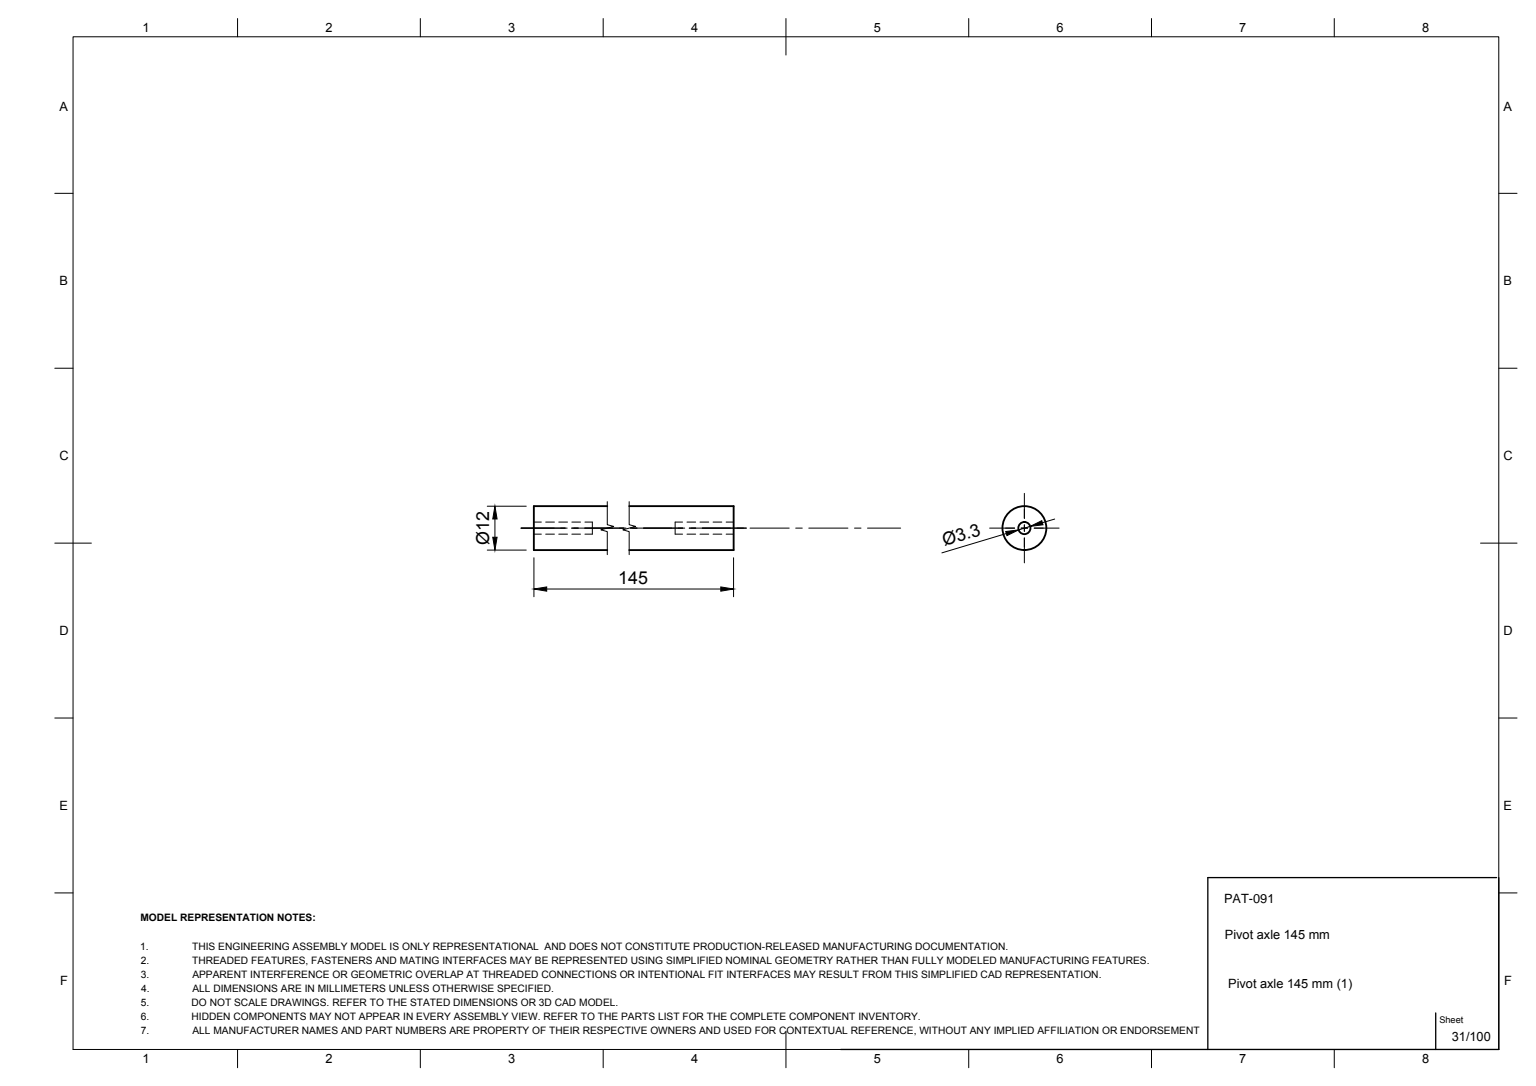
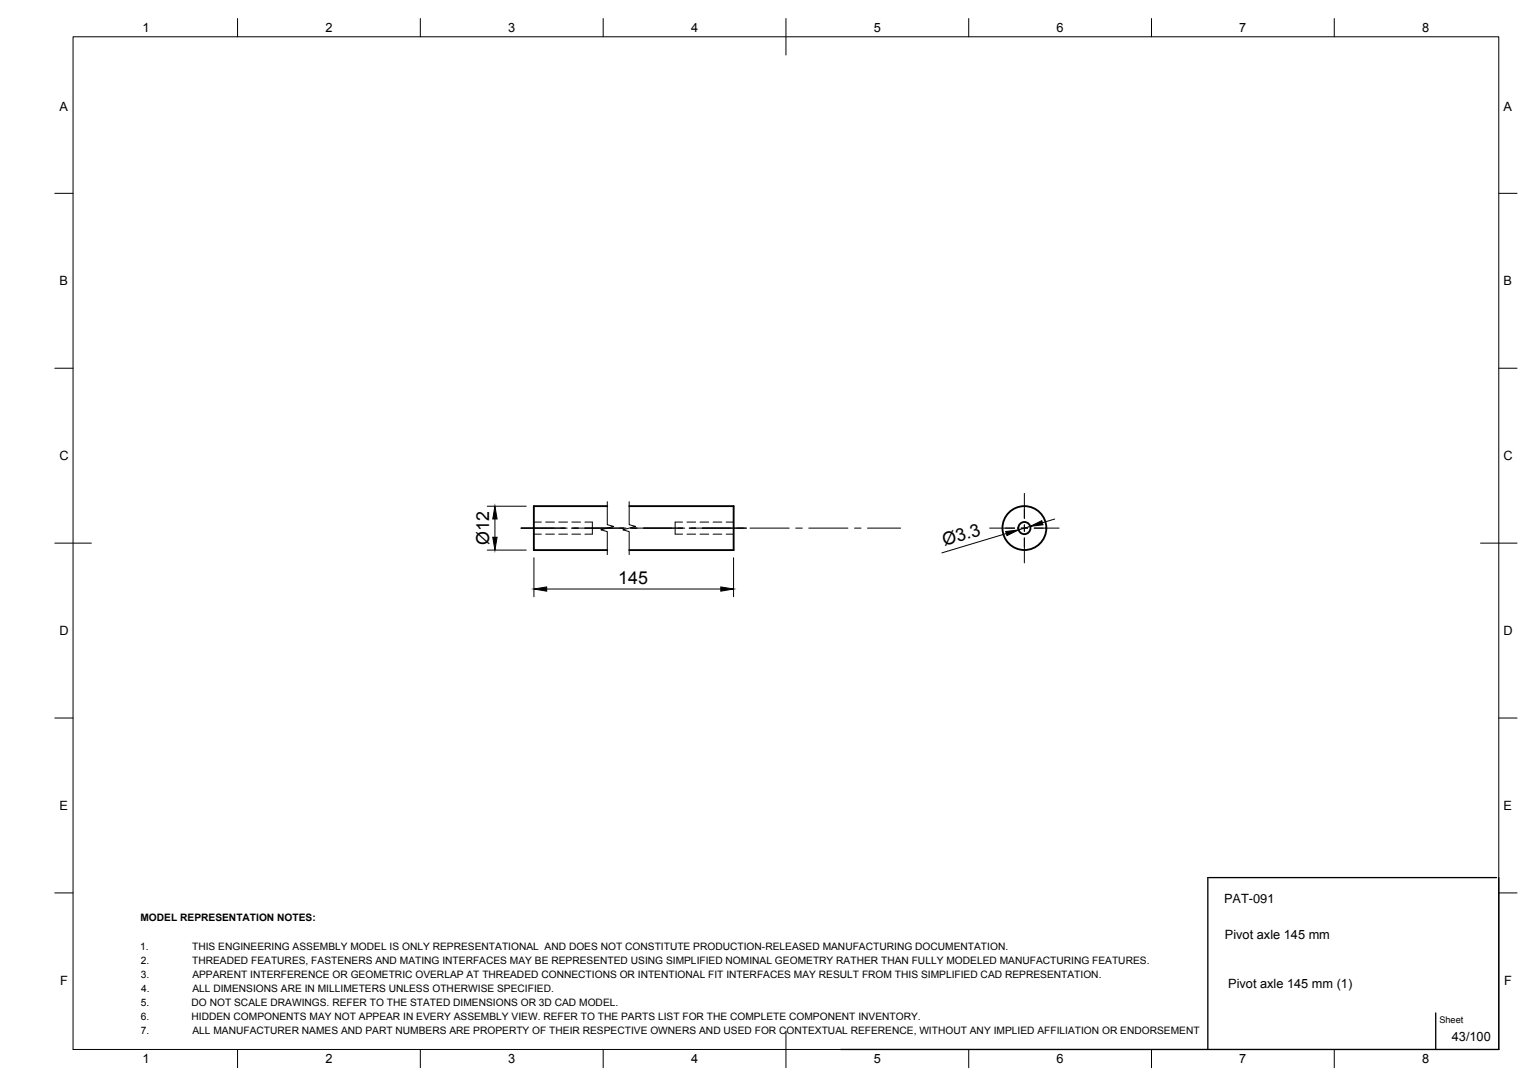
ISO-10303-21;
HEADER;
/* Generated by software containing ST-Developer
 * from STEP Tools, Inc. (www.steptools.com) 
 */

FILE_DESCRIPTION(
/* description */ ('PAT-091'),
/* implementation_level */ '2;1');

FILE_NAME(
/* name */ 'Pivot axle 145 mm.step',
/* time_stamp */ '2026-10-27T15:34:44-07:00',
/* author */ (''),
/* organization */ (''),
/* preprocessor_version */ 'ST-DEVELOPER v20.2',
/* originating_system */ 'Autodesk Translation Framework v15.17.0.0',
/* authorisation */ '');

FILE_SCHEMA (('AUTOMOTIVE_DESIGN { 1 0 10303 214 3 1 1 }'));
ENDSEC;

DATA;
#10=MECHANICAL_DESIGN_GEOMETRIC_PRESENTATION_REPRESENTATION('',(#994),#25100);
#774=SHAPE_REPRESENTATION_RELATIONSHIP('SRR','None',#25536,#884);
#884=ADVANCED_BREP_SHAPE_REPRESENTATION('',(#1117),#25006);
#994=STYLED_ITEM('',(#26191),#1117);
#1117=MANIFOLD_SOLID_BREP('Body1',#13272);
#1377=FACE_BOUND('',#3261,.T.);
#1378=FACE_BOUND('',#3263,.T.);
#1750=PLANE('',#15028);
#1751=PLANE('',#15032);
#1752=PLANE('',#15036);
#1753=PLANE('',#15037);
#2275=FACE_OUTER_BOUND('',#3255,.T.);
#2276=FACE_OUTER_BOUND('',#3256,.T.);
#2277=FACE_OUTER_BOUND('',#3257,.T.);
#2278=FACE_OUTER_BOUND('',#3258,.T.);
#2279=FACE_OUTER_BOUND('',#3259,.T.);
#2280=FACE_OUTER_BOUND('',#3260,.T.);
#2281=FACE_OUTER_BOUND('',#3262,.T.);
#3255=EDGE_LOOP('',(#9902,#9903,#9904,#9905));
#3256=EDGE_LOOP('',(#9906));
#3257=EDGE_LOOP('',(#9907,#9908,#9909,#9910));
#3258=EDGE_LOOP('',(#9911));
#3259=EDGE_LOOP('',(#9912,#9913,#9914,#9915));
#3260=EDGE_LOOP('',(#9916));
#3261=EDGE_LOOP('',(#9917));
#3262=EDGE_LOOP('',(#9918));
#3263=EDGE_LOOP('',(#9919));
#4388=LINE('',#21991,#5128);
#4389=LINE('',#21998,#5129);
#4390=LINE('',#22005,#5130);
#5128=VECTOR('',#17616,0.165);
#5129=VECTOR('',#17625,0.165);
#5130=VECTOR('',#17634,0.6);
#5805=CIRCLE('',#15026,0.165);
#5806=CIRCLE('',#15027,0.165);
#5807=CIRCLE('',#15030,0.165);
#5808=CIRCLE('',#15031,0.165);
#5809=CIRCLE('',#15034,0.6);
#5810=CIRCLE('',#15035,0.6);
#6692=VERTEX_POINT('',#21988);
#6693=VERTEX_POINT('',#21990);
#6694=VERTEX_POINT('',#21995);
#6695=VERTEX_POINT('',#21997);
#6696=VERTEX_POINT('',#22002);
#6697=VERTEX_POINT('',#22004);
#7886=EDGE_CURVE('',#6692,#6692,#5805,.T.);
#7887=EDGE_CURVE('',#6692,#6693,#4388,.T.);
#7888=EDGE_CURVE('',#6693,#6693,#5806,.T.);
#7889=EDGE_CURVE('',#6694,#6694,#5807,.T.);
#7890=EDGE_CURVE('',#6694,#6695,#4389,.T.);
#7891=EDGE_CURVE('',#6695,#6695,#5808,.T.);
#7892=EDGE_CURVE('',#6696,#6696,#5809,.T.);
#7893=EDGE_CURVE('',#6696,#6697,#4390,.T.);
#7894=EDGE_CURVE('',#6697,#6697,#5810,.T.);
#9902=ORIENTED_EDGE('',*,*,#7886,.F.);
#9903=ORIENTED_EDGE('',*,*,#7887,.T.);
#9904=ORIENTED_EDGE('',*,*,#7888,.F.);
#9905=ORIENTED_EDGE('',*,*,#7887,.F.);
#9906=ORIENTED_EDGE('',*,*,#7886,.T.);
#9907=ORIENTED_EDGE('',*,*,#7889,.F.);
#9908=ORIENTED_EDGE('',*,*,#7890,.T.);
#9909=ORIENTED_EDGE('',*,*,#7891,.T.);
#9910=ORIENTED_EDGE('',*,*,#7890,.F.);
#9911=ORIENTED_EDGE('',*,*,#7891,.F.);
#9912=ORIENTED_EDGE('',*,*,#7892,.F.);
#9913=ORIENTED_EDGE('',*,*,#7893,.T.);
#9914=ORIENTED_EDGE('',*,*,#7894,.T.);
#9915=ORIENTED_EDGE('',*,*,#7893,.F.);
#9916=ORIENTED_EDGE('',*,*,#7892,.T.);
#9917=ORIENTED_EDGE('',*,*,#7888,.T.);
#9918=ORIENTED_EDGE('',*,*,#7894,.F.);
#9919=ORIENTED_EDGE('',*,*,#7889,.T.);
#12173=CYLINDRICAL_SURFACE('',#15025,0.165);
#12174=CYLINDRICAL_SURFACE('',#15029,0.165);
#12175=CYLINDRICAL_SURFACE('',#15033,0.6);
#12642=ADVANCED_FACE('',(#2275),#12173,.F.);
#12643=ADVANCED_FACE('',(#2276),#1750,.T.);
#12644=ADVANCED_FACE('',(#2277),#12174,.F.);
#12645=ADVANCED_FACE('',(#2278),#1751,.F.);
#12646=ADVANCED_FACE('',(#2279),#12175,.T.);
#12647=ADVANCED_FACE('',(#2280,#1377),#1752,.T.);
#12648=ADVANCED_FACE('',(#2281,#1378),#1753,.F.);
#13272=CLOSED_SHELL('',(#12642,#12643,#12644,#12645,#12646,#12647,#12648));
#15024=AXIS2_PLACEMENT_3D('',#21986,#17610,#17611);
#15025=AXIS2_PLACEMENT_3D('',#21987,#17612,#17613);
#15026=AXIS2_PLACEMENT_3D('',#21989,#17614,#17615);
#15027=AXIS2_PLACEMENT_3D('',#21992,#17617,#17618);
#15028=AXIS2_PLACEMENT_3D('',#21993,#17619,#17620);
#15029=AXIS2_PLACEMENT_3D('',#21994,#17621,#17622);
#15030=AXIS2_PLACEMENT_3D('',#21996,#17623,#17624);
#15031=AXIS2_PLACEMENT_3D('',#21999,#17626,#17627);
#15032=AXIS2_PLACEMENT_3D('',#22000,#17628,#17629);
#15033=AXIS2_PLACEMENT_3D('',#22001,#17630,#17631);
#15034=AXIS2_PLACEMENT_3D('',#22003,#17632,#17633);
#15035=AXIS2_PLACEMENT_3D('',#22006,#17635,#17636);
#15036=AXIS2_PLACEMENT_3D('',#22007,#17637,#17638);
#15037=AXIS2_PLACEMENT_3D('',#22008,#17639,#17640);
#17610=DIRECTION('axis',(0.,0.,1.));
#17611=DIRECTION('refdir',(1.,0.,0.));
#17612=DIRECTION('center_axis',(0.,1.,0.));
#17613=DIRECTION('ref_axis',(1.,0.,0.));
#17614=DIRECTION('center_axis',(0.,1.,0.));
#17615=DIRECTION('ref_axis',(1.,0.,0.));
#17616=DIRECTION('',(0.,1.,0.));
#17617=DIRECTION('center_axis',(0.,-1.,0.));
#17618=DIRECTION('ref_axis',(1.,0.,0.));
#17619=DIRECTION('center_axis',(0.,1.,0.));
#17620=DIRECTION('ref_axis',(1.,0.,0.));
#17621=DIRECTION('center_axis',(0.,1.,0.));
#17622=DIRECTION('ref_axis',(1.,0.,0.));
#17623=DIRECTION('center_axis',(0.,1.,0.));
#17624=DIRECTION('ref_axis',(1.,0.,0.));
#17625=DIRECTION('',(0.,1.,0.));
#17626=DIRECTION('center_axis',(0.,1.,0.));
#17627=DIRECTION('ref_axis',(1.,0.,0.));
#17628=DIRECTION('center_axis',(0.,1.,0.));
#17629=DIRECTION('ref_axis',(1.,0.,0.));
#17630=DIRECTION('center_axis',(0.,1.,0.));
#17631=DIRECTION('ref_axis',(1.,0.,0.));
#17632=DIRECTION('center_axis',(0.,1.,0.));
#17633=DIRECTION('ref_axis',(1.,0.,0.));
#17634=DIRECTION('',(0.,-1.,0.));
#17635=DIRECTION('center_axis',(0.,1.,0.));
#17636=DIRECTION('ref_axis',(1.,0.,0.));
#17637=DIRECTION('center_axis',(0.,1.,0.));
#17638=DIRECTION('ref_axis',(1.,0.,0.));
#17639=DIRECTION('center_axis',(0.,1.,0.));
#17640=DIRECTION('ref_axis',(1.,0.,0.));
#21986=CARTESIAN_POINT('',(0.,0.,0.));
#21987=CARTESIAN_POINT('Origin',(0.,6.9,13.));
#21988=CARTESIAN_POINT('',(-0.165,6.9,13.));
#21989=CARTESIAN_POINT('Origin',(0.,6.9,13.));
#21990=CARTESIAN_POINT('',(-0.165,8.5,13.));
#21991=CARTESIAN_POINT('',(-0.165,6.9,13.));
#21992=CARTESIAN_POINT('Origin',(0.,8.5,13.));
#21993=CARTESIAN_POINT('Origin',(0.,6.9,13.));
#21994=CARTESIAN_POINT('Origin',(0.,-6.1,13.));
#21995=CARTESIAN_POINT('',(-0.165,-6.,13.));
#21996=CARTESIAN_POINT('Origin',(0.,-6.,13.));
#21997=CARTESIAN_POINT('',(-0.165,-4.4,13.));
#21998=CARTESIAN_POINT('',(-0.165,-6.1,13.));
#21999=CARTESIAN_POINT('Origin',(0.,-4.4,13.));
#22000=CARTESIAN_POINT('Origin',(0.,-4.4,13.));
#22001=CARTESIAN_POINT('Origin',(0.,-6.,13.));
#22002=CARTESIAN_POINT('',(-0.6,8.5,13.));
#22003=CARTESIAN_POINT('Origin',(0.,8.5,13.));
#22004=CARTESIAN_POINT('',(-0.6,-6.,13.));
#22005=CARTESIAN_POINT('',(-0.6,-6.,13.));
#22006=CARTESIAN_POINT('Origin',(0.,-6.,13.));
#22007=CARTESIAN_POINT('Origin',(0.,8.5,13.));
#22008=CARTESIAN_POINT('Origin',(0.,-6.,13.));
#24885=UNCERTAINTY_MEASURE_WITH_UNIT(LENGTH_MEASURE(0.001),#25101,
'DISTANCE_ACCURACY_VALUE',
'Maximum model space distance between geometric entities at asserted c
onnectivities');
#24979=UNCERTAINTY_MEASURE_WITH_UNIT(LENGTH_MEASURE(0.001),#25101,
'DISTANCE_ACCURACY_VALUE',
'Maximum model space distance between geometric entities at asserted c
onnectivities');
#25006=(
GEOMETRIC_REPRESENTATION_CONTEXT(3)
GLOBAL_UNCERTAINTY_ASSIGNED_CONTEXT((#24885))
GLOBAL_UNIT_ASSIGNED_CONTEXT((#25101,#25103,#25104))
REPRESENTATION_CONTEXT('','3D')
);
#25100=(
GEOMETRIC_REPRESENTATION_CONTEXT(3)
GLOBAL_UNCERTAINTY_ASSIGNED_CONTEXT((#24979))
GLOBAL_UNIT_ASSIGNED_CONTEXT((#25101,#25103,#25104))
REPRESENTATION_CONTEXT('','3D')
);
#25101=(
LENGTH_UNIT()
NAMED_UNIT(*)
SI_UNIT(.CENTI.,.METRE.)
);
#25103=(
NAMED_UNIT(*)
PLANE_ANGLE_UNIT()
SI_UNIT($,.RADIAN.)
);
#25104=(
NAMED_UNIT(*)
SI_UNIT($,.STERADIAN.)
SOLID_ANGLE_UNIT()
);
#25131=SHAPE_DEFINITION_REPRESENTATION(#25251,#25536);
#25251=PRODUCT_DEFINITION_SHAPE('',$,#25657);
#25536=SHAPE_REPRESENTATION('',(#15024),#25006);
#25630=PRODUCT_DEFINITION_CONTEXT('part definition',#25992,'design');
#25657=PRODUCT_DEFINITION('Pivot axle 145 mm','Pivot axle 145 mm',#25777,
#25630);
#25777=PRODUCT_DEFINITION_FORMATION('',$,#26020);
#25992=APPLICATION_CONTEXT(
'Core Data for Automotive Mechanical Design Process');
#25993=PRODUCT_CONTEXT('part definition',#25992,'mechanical');
#26020=PRODUCT('Pivot axle 145 mm','Pivot axle 145 mm',
'Pivot axle 145 mm',(#25993));
#26185=COLOUR_RGB('Grey',0.48,0.52,0.57);
#26186=FILL_AREA_STYLE_COLOUR('',#26185);
#26187=FILL_AREA_STYLE('',(#26186));
#26188=SURFACE_STYLE_FILL_AREA(#26187);
#26189=SURFACE_SIDE_STYLE('',(#26188));
#26190=SURFACE_STYLE_USAGE(.BOTH.,#26189);
#26191=PRESENTATION_STYLE_ASSIGNMENT((#26190));
ENDSEC;
END-ISO-10303-21;
